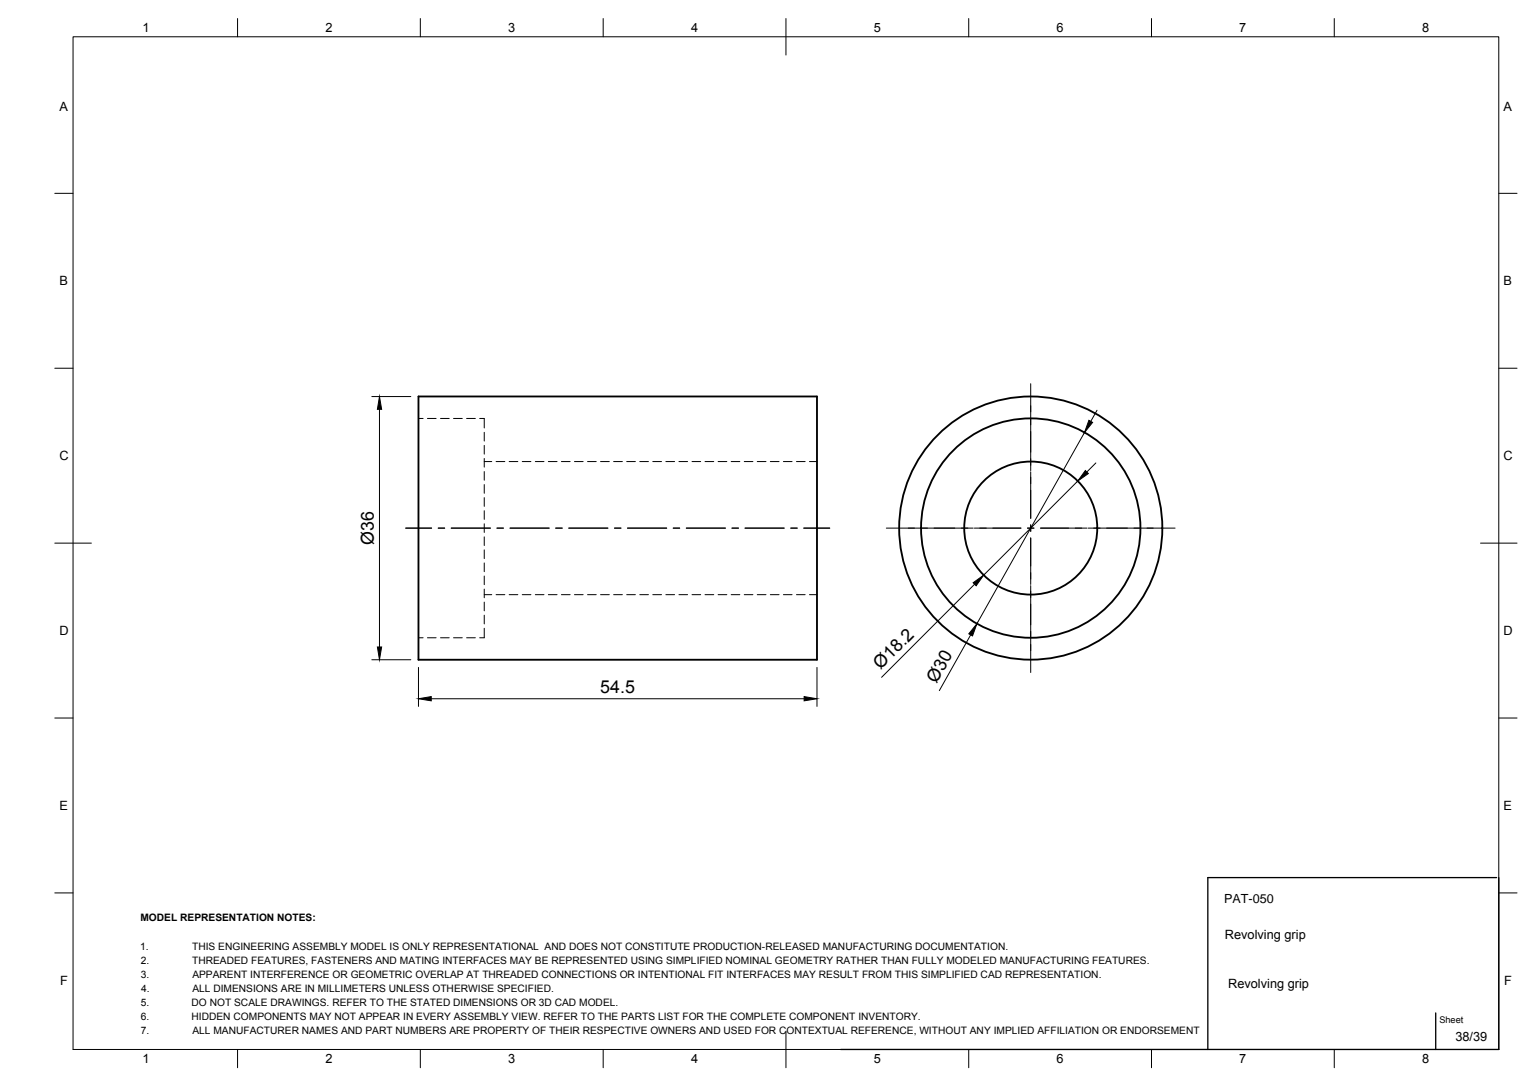
ISO-10303-21;
HEADER;
/* Generated by software containing ST-Developer
 * from STEP Tools, Inc. (www.steptools.com) 
 */

FILE_DESCRIPTION(
/* description */ ('Hand wheel with handle and shaft collar'),
/* implementation_level */ '2;1');

FILE_NAME(
/* name */ 'Revolving grip.step',
/* time_stamp */ '2026-10-28T03:23:19-07:00',
/* author */ (''),
/* organization */ (''),
/* preprocessor_version */ 'ST-DEVELOPER v20.2',
/* originating_system */ 'Autodesk Translation Framework v15.17.0.0',
/* authorisation */ '');

FILE_SCHEMA (('AUTOMOTIVE_DESIGN { 1 0 10303 214 3 1 1 }'));
ENDSEC;

DATA;
#10=MECHANICAL_DESIGN_GEOMETRIC_PRESENTATION_REPRESENTATION('',(#440),#10510);
#361=SHAPE_REPRESENTATION_RELATIONSHIP('SRR','None',#10681,#393);
#393=ADVANCED_BREP_SHAPE_REPRESENTATION('',(#484),#10508);
#440=STYLED_ITEM('',(#10915),#484);
#484=MANIFOLD_SOLID_BREP('Body1',#5342);
#593=FACE_BOUND('',#1500,.T.);
#594=FACE_BOUND('',#1504,.T.);
#595=FACE_BOUND('',#1506,.T.);
#758=PLANE('',#6396);
#759=PLANE('',#6403);
#760=PLANE('',#6404);
#1072=FACE_OUTER_BOUND('',#1498,.T.);
#1073=FACE_OUTER_BOUND('',#1499,.T.);
#1074=FACE_OUTER_BOUND('',#1501,.T.);
#1075=FACE_OUTER_BOUND('',#1502,.T.);
#1076=FACE_OUTER_BOUND('',#1503,.T.);
#1077=FACE_OUTER_BOUND('',#1505,.T.);
#1498=EDGE_LOOP('',(#4849,#4850,#4851,#4852));
#1499=EDGE_LOOP('',(#4853));
#1500=EDGE_LOOP('',(#4854));
#1501=EDGE_LOOP('',(#4855,#4856,#4857,#4858));
#1502=EDGE_LOOP('',(#4859,#4860,#4861,#4862));
#1503=EDGE_LOOP('',(#4863));
#1504=EDGE_LOOP('',(#4864));
#1505=EDGE_LOOP('',(#4865));
#1506=EDGE_LOOP('',(#4866));
#1818=LINE('',#10396,#2128);
#1819=LINE('',#10403,#2129);
#1820=LINE('',#10409,#2130);
#2128=VECTOR('',#8120,1.5);
#2129=VECTOR('',#8129,0.91);
#2130=VECTOR('',#8136,1.8);
#2434=CIRCLE('',#6394,1.5);
#2435=CIRCLE('',#6395,1.5);
#2436=CIRCLE('',#6397,0.91);
#2437=CIRCLE('',#6399,0.91);
#2438=CIRCLE('',#6401,1.8);
#2439=CIRCLE('',#6402,1.8);
#2886=VERTEX_POINT('',#10393);
#2887=VERTEX_POINT('',#10395);
#2888=VERTEX_POINT('',#10399);
#2889=VERTEX_POINT('',#10402);
#2890=VERTEX_POINT('',#10406);
#2891=VERTEX_POINT('',#10408);
#3542=EDGE_CURVE('',#2886,#2886,#2434,.T.);
#3543=EDGE_CURVE('',#2886,#2887,#1818,.T.);
#3544=EDGE_CURVE('',#2887,#2887,#2435,.T.);
#3545=EDGE_CURVE('',#2888,#2888,#2436,.T.);
#3546=EDGE_CURVE('',#2888,#2889,#1819,.T.);
#3547=EDGE_CURVE('',#2889,#2889,#2437,.T.);
#3548=EDGE_CURVE('',#2890,#2890,#2438,.T.);
#3549=EDGE_CURVE('',#2890,#2891,#1820,.T.);
#3550=EDGE_CURVE('',#2891,#2891,#2439,.T.);
#4849=ORIENTED_EDGE('',*,*,#3542,.F.);
#4850=ORIENTED_EDGE('',*,*,#3543,.T.);
#4851=ORIENTED_EDGE('',*,*,#3544,.F.);
#4852=ORIENTED_EDGE('',*,*,#3543,.F.);
#4853=ORIENTED_EDGE('',*,*,#3542,.T.);
#4854=ORIENTED_EDGE('',*,*,#3545,.F.);
#4855=ORIENTED_EDGE('',*,*,#3545,.T.);
#4856=ORIENTED_EDGE('',*,*,#3546,.T.);
#4857=ORIENTED_EDGE('',*,*,#3547,.T.);
#4858=ORIENTED_EDGE('',*,*,#3546,.F.);
#4859=ORIENTED_EDGE('',*,*,#3548,.F.);
#4860=ORIENTED_EDGE('',*,*,#3549,.T.);
#4861=ORIENTED_EDGE('',*,*,#3550,.T.);
#4862=ORIENTED_EDGE('',*,*,#3549,.F.);
#4863=ORIENTED_EDGE('',*,*,#3548,.T.);
#4864=ORIENTED_EDGE('',*,*,#3544,.T.);
#4865=ORIENTED_EDGE('',*,*,#3550,.F.);
#4866=ORIENTED_EDGE('',*,*,#3547,.F.);
#4970=CYLINDRICAL_SURFACE('',#6393,1.5);
#4971=CYLINDRICAL_SURFACE('',#6398,0.91);
#4972=CYLINDRICAL_SURFACE('',#6400,1.8);
#5284=ADVANCED_FACE('',(#1072),#4970,.F.);
#5285=ADVANCED_FACE('',(#1073,#593),#758,.T.);
#5286=ADVANCED_FACE('',(#1074),#4971,.F.);
#5287=ADVANCED_FACE('',(#1075),#4972,.T.);
#5288=ADVANCED_FACE('',(#1076,#594),#759,.T.);
#5289=ADVANCED_FACE('',(#1077,#595),#760,.F.);
#5342=CLOSED_SHELL('',(#5284,#5285,#5286,#5287,#5288,#5289));
#6392=AXIS2_PLACEMENT_3D('',#10391,#8114,#8115);
#6393=AXIS2_PLACEMENT_3D('',#10392,#8116,#8117);
#6394=AXIS2_PLACEMENT_3D('',#10394,#8118,#8119);
#6395=AXIS2_PLACEMENT_3D('',#10397,#8121,#8122);
#6396=AXIS2_PLACEMENT_3D('',#10398,#8123,#8124);
#6397=AXIS2_PLACEMENT_3D('',#10400,#8125,#8126);
#6398=AXIS2_PLACEMENT_3D('',#10401,#8127,#8128);
#6399=AXIS2_PLACEMENT_3D('',#10404,#8130,#8131);
#6400=AXIS2_PLACEMENT_3D('',#10405,#8132,#8133);
#6401=AXIS2_PLACEMENT_3D('',#10407,#8134,#8135);
#6402=AXIS2_PLACEMENT_3D('',#10410,#8137,#8138);
#6403=AXIS2_PLACEMENT_3D('',#10411,#8139,#8140);
#6404=AXIS2_PLACEMENT_3D('',#10412,#8141,#8142);
#8114=DIRECTION('axis',(0.,0.,1.));
#8115=DIRECTION('refdir',(1.,0.,0.));
#8116=DIRECTION('center_axis',(0.,1.,0.));
#8117=DIRECTION('ref_axis',(1.,0.,0.));
#8118=DIRECTION('center_axis',(0.,1.,0.));
#8119=DIRECTION('ref_axis',(1.,0.,0.));
#8120=DIRECTION('',(0.,1.,0.));
#8121=DIRECTION('center_axis',(0.,-1.,0.));
#8122=DIRECTION('ref_axis',(1.,0.,0.));
#8123=DIRECTION('center_axis',(0.,1.,0.));
#8124=DIRECTION('ref_axis',(1.,0.,0.));
#8125=DIRECTION('center_axis',(0.,1.,0.));
#8126=DIRECTION('ref_axis',(1.,0.,0.));
#8127=DIRECTION('center_axis',(0.,1.,0.));
#8128=DIRECTION('ref_axis',(1.,0.,0.));
#8129=DIRECTION('',(0.,-1.,0.));
#8130=DIRECTION('center_axis',(0.,-1.,0.));
#8131=DIRECTION('ref_axis',(1.,0.,0.));
#8132=DIRECTION('center_axis',(0.,1.,0.));
#8133=DIRECTION('ref_axis',(1.,0.,0.));
#8134=DIRECTION('center_axis',(0.,1.,0.));
#8135=DIRECTION('ref_axis',(1.,0.,0.));
#8136=DIRECTION('',(0.,-1.,0.));
#8137=DIRECTION('center_axis',(0.,1.,0.));
#8138=DIRECTION('ref_axis',(1.,0.,0.));
#8139=DIRECTION('center_axis',(0.,1.,0.));
#8140=DIRECTION('ref_axis',(1.,0.,0.));
#8141=DIRECTION('center_axis',(0.,1.,0.));
#8142=DIRECTION('ref_axis',(1.,0.,0.));
#10391=CARTESIAN_POINT('',(0.,0.,0.));
#10392=CARTESIAN_POINT('Origin',(6.5,-5.45,10.));
#10393=CARTESIAN_POINT('',(5.,-5.45,10.));
#10394=CARTESIAN_POINT('Origin',(6.5,-5.45,10.));
#10395=CARTESIAN_POINT('',(5.,-4.55,10.));
#10396=CARTESIAN_POINT('',(5.,-5.45,10.));
#10397=CARTESIAN_POINT('Origin',(6.5,-4.55,10.));
#10398=CARTESIAN_POINT('Origin',(6.5,-5.45,10.));
#10399=CARTESIAN_POINT('',(5.59,-5.45,10.));
#10400=CARTESIAN_POINT('Origin',(6.5,-5.45,10.));
#10401=CARTESIAN_POINT('Origin',(6.5,-10.,10.));
#10402=CARTESIAN_POINT('',(5.59,-10.,10.));
#10403=CARTESIAN_POINT('',(5.59,-10.,10.));
#10404=CARTESIAN_POINT('Origin',(6.5,-10.,10.));
#10405=CARTESIAN_POINT('Origin',(6.5,-10.,10.));
#10406=CARTESIAN_POINT('',(4.7,-4.55,10.));
#10407=CARTESIAN_POINT('Origin',(6.5,-4.55,10.));
#10408=CARTESIAN_POINT('',(4.7,-10.,10.));
#10409=CARTESIAN_POINT('',(4.7,-10.,10.));
#10410=CARTESIAN_POINT('Origin',(6.5,-10.,10.));
#10411=CARTESIAN_POINT('Origin',(6.5,-4.55,10.));
#10412=CARTESIAN_POINT('Origin',(6.5,-10.,10.));
#10469=UNCERTAINTY_MEASURE_WITH_UNIT(LENGTH_MEASURE(0.001),#10511,
'DISTANCE_ACCURACY_VALUE',
'Maximum model space distance between geometric entities at asserted c
onnectivities');
#10471=UNCERTAINTY_MEASURE_WITH_UNIT(LENGTH_MEASURE(0.001),#10511,
'DISTANCE_ACCURACY_VALUE',
'Maximum model space distance between geometric entities at asserted c
onnectivities');
#10508=(
GEOMETRIC_REPRESENTATION_CONTEXT(3)
GLOBAL_UNCERTAINTY_ASSIGNED_CONTEXT((#10469))
GLOBAL_UNIT_ASSIGNED_CONTEXT((#10511,#10513,#10514))
REPRESENTATION_CONTEXT('','3D')
);
#10510=(
GEOMETRIC_REPRESENTATION_CONTEXT(3)
GLOBAL_UNCERTAINTY_ASSIGNED_CONTEXT((#10471))
GLOBAL_UNIT_ASSIGNED_CONTEXT((#10511,#10513,#10514))
REPRESENTATION_CONTEXT('','3D')
);
#10511=(
LENGTH_UNIT()
NAMED_UNIT(*)
SI_UNIT(.CENTI.,.METRE.)
);
#10513=(
NAMED_UNIT(*)
PLANE_ANGLE_UNIT()
SI_UNIT($,.RADIAN.)
);
#10514=(
NAMED_UNIT(*)
SI_UNIT($,.STERADIAN.)
SOLID_ANGLE_UNIT()
);
#10551=SHAPE_DEFINITION_REPRESENTATION(#10638,#10681);
#10638=PRODUCT_DEFINITION_SHAPE('',$,#10720);
#10681=SHAPE_REPRESENTATION('',(#6392),#10508);
#10683=PRODUCT_DEFINITION_CONTEXT('part definition',#10799,'design');
#10720=PRODUCT_DEFINITION('Revolving grip','Revolving grip',#10758,#10683);
#10758=PRODUCT_DEFINITION_FORMATION('',$,#10837);
#10799=APPLICATION_CONTEXT(
'Core Data for Automotive Mechanical Design Process');
#10800=PRODUCT_CONTEXT('part definition',#10799,'mechanical');
#10837=PRODUCT('Revolving grip','Revolving grip','Revolving grip',(#10800));
#10909=COLOUR_RGB('Black',0.12,0.14,0.17);
#10910=FILL_AREA_STYLE_COLOUR('',#10909);
#10911=FILL_AREA_STYLE('',(#10910));
#10912=SURFACE_STYLE_FILL_AREA(#10911);
#10913=SURFACE_SIDE_STYLE('',(#10912));
#10914=SURFACE_STYLE_USAGE(.BOTH.,#10913);
#10915=PRESENTATION_STYLE_ASSIGNMENT((#10914));
ENDSEC;
END-ISO-10303-21;
